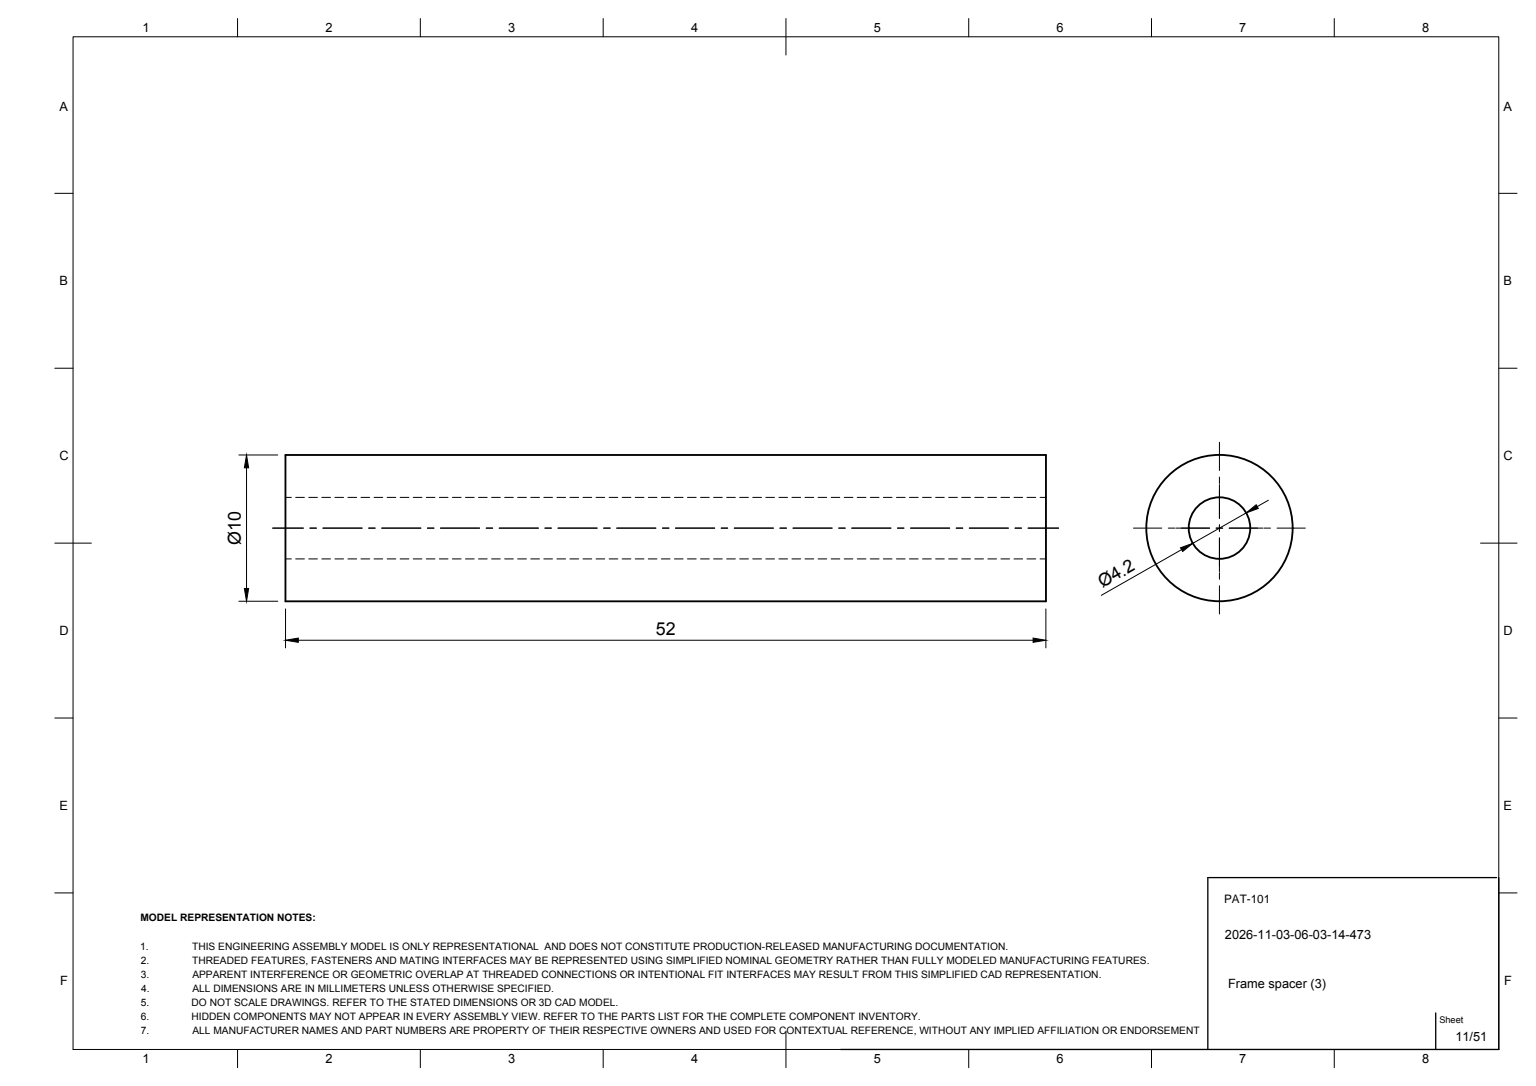
ISO-10303-21;
HEADER;
/* Generated by software containing ST-Developer
 * from STEP Tools, Inc. (www.steptools.com) 
 */

FILE_DESCRIPTION(
/* description */ ('Spur gear reduction stage 2-1 on bearing plates'),
/* implementation_level */ '2;1');

FILE_NAME(
/* name */ 'Frame spacer (3).step',
/* time_stamp */ '2026-10-28T03:22:07-07:00',
/* author */ (''),
/* organization */ (''),
/* preprocessor_version */ 'ST-DEVELOPER v20.2',
/* originating_system */ 'Autodesk Translation Framework v15.17.0.0',
/* authorisation */ '');

FILE_SCHEMA (('AUTOMOTIVE_DESIGN { 1 0 10303 214 3 1 1 }'));
ENDSEC;

DATA;
#10=MECHANICAL_DESIGN_GEOMETRIC_PRESENTATION_REPRESENTATION('',(#953),#53909);
#867=SHAPE_REPRESENTATION_RELATIONSHIP('SRR','None',#54094,#910);
#910=ADVANCED_BREP_SHAPE_REPRESENTATION('',(#1011),#53868);
#953=STYLED_ITEM('',(#54376),#1011);
#1011=MANIFOLD_SOLID_BREP('Body1',#11277);
#1138=FACE_BOUND('',#2322,.T.);
#1139=FACE_BOUND('',#2324,.T.);
#1278=PLANE('',#12011);
#1279=PLANE('',#12012);
#1593=FACE_OUTER_BOUND('',#2319,.T.);
#1594=FACE_OUTER_BOUND('',#2320,.T.);
#1595=FACE_OUTER_BOUND('',#2321,.T.);
#1596=FACE_OUTER_BOUND('',#2323,.T.);
#2319=EDGE_LOOP('',(#7724,#7725,#7726,#7727));
#2320=EDGE_LOOP('',(#7728,#7729,#7730,#7731));
#2321=EDGE_LOOP('',(#7732));
#2322=EDGE_LOOP('',(#7733));
#2323=EDGE_LOOP('',(#7734));
#2324=EDGE_LOOP('',(#7735));
#3063=LINE('',#16388,#3704);
#3064=LINE('',#16394,#3705);
#3704=VECTOR('',#13470,0.210000000000001);
#3705=VECTOR('',#13477,0.5);
#4359=CIRCLE('',#12006,0.210000000000001);
#4360=CIRCLE('',#12007,0.210000000000001);
#4361=CIRCLE('',#12009,0.5);
#4362=CIRCLE('',#12010,0.5);
#4908=VERTEX_POINT('',#16385);
#4909=VERTEX_POINT('',#16387);
#4910=VERTEX_POINT('',#16391);
#4911=VERTEX_POINT('',#16393);
#6004=EDGE_CURVE('',#4908,#4908,#4359,.T.);
#6005=EDGE_CURVE('',#4908,#4909,#3063,.T.);
#6006=EDGE_CURVE('',#4909,#4909,#4360,.T.);
#6007=EDGE_CURVE('',#4910,#4910,#4361,.T.);
#6008=EDGE_CURVE('',#4910,#4911,#3064,.T.);
#6009=EDGE_CURVE('',#4911,#4911,#4362,.T.);
#7724=ORIENTED_EDGE('',*,*,#6004,.F.);
#7725=ORIENTED_EDGE('',*,*,#6005,.T.);
#7726=ORIENTED_EDGE('',*,*,#6006,.T.);
#7727=ORIENTED_EDGE('',*,*,#6005,.F.);
#7728=ORIENTED_EDGE('',*,*,#6007,.F.);
#7729=ORIENTED_EDGE('',*,*,#6008,.T.);
#7730=ORIENTED_EDGE('',*,*,#6009,.T.);
#7731=ORIENTED_EDGE('',*,*,#6008,.F.);
#7732=ORIENTED_EDGE('',*,*,#6007,.T.);
#7733=ORIENTED_EDGE('',*,*,#6004,.T.);
#7734=ORIENTED_EDGE('',*,*,#6009,.F.);
#7735=ORIENTED_EDGE('',*,*,#6006,.F.);
#10470=CYLINDRICAL_SURFACE('',#12005,0.210000000000001);
#10471=CYLINDRICAL_SURFACE('',#12008,0.5);
#10713=ADVANCED_FACE('',(#1593),#10470,.F.);
#10714=ADVANCED_FACE('',(#1594),#10471,.T.);
#10715=ADVANCED_FACE('',(#1595,#1138),#1278,.T.);
#10716=ADVANCED_FACE('',(#1596,#1139),#1279,.F.);
#11277=CLOSED_SHELL('',(#10713,#10714,#10715,#10716));
#12004=AXIS2_PLACEMENT_3D('',#16383,#13464,#13465);
#12005=AXIS2_PLACEMENT_3D('',#16384,#13466,#13467);
#12006=AXIS2_PLACEMENT_3D('',#16386,#13468,#13469);
#12007=AXIS2_PLACEMENT_3D('',#16389,#13471,#13472);
#12008=AXIS2_PLACEMENT_3D('',#16390,#13473,#13474);
#12009=AXIS2_PLACEMENT_3D('',#16392,#13475,#13476);
#12010=AXIS2_PLACEMENT_3D('',#16395,#13478,#13479);
#12011=AXIS2_PLACEMENT_3D('',#16396,#13480,#13481);
#12012=AXIS2_PLACEMENT_3D('',#16397,#13482,#13483);
#13464=DIRECTION('axis',(0.,0.,1.));
#13465=DIRECTION('refdir',(1.,0.,0.));
#13466=DIRECTION('center_axis',(0.,1.,0.));
#13467=DIRECTION('ref_axis',(1.,0.,0.));
#13468=DIRECTION('center_axis',(0.,-1.,0.));
#13469=DIRECTION('ref_axis',(1.,0.,0.));
#13470=DIRECTION('',(0.,-1.,0.));
#13471=DIRECTION('center_axis',(0.,-1.,0.));
#13472=DIRECTION('ref_axis',(1.,0.,0.));
#13473=DIRECTION('center_axis',(0.,1.,0.));
#13474=DIRECTION('ref_axis',(1.,0.,0.));
#13475=DIRECTION('center_axis',(0.,1.,0.));
#13476=DIRECTION('ref_axis',(1.,0.,0.));
#13477=DIRECTION('',(0.,-1.,0.));
#13478=DIRECTION('center_axis',(0.,1.,0.));
#13479=DIRECTION('ref_axis',(1.,0.,0.));
#13480=DIRECTION('center_axis',(0.,1.,0.));
#13481=DIRECTION('ref_axis',(1.,0.,0.));
#13482=DIRECTION('center_axis',(0.,1.,0.));
#13483=DIRECTION('ref_axis',(1.,0.,0.));
#16383=CARTESIAN_POINT('',(0.,0.,0.));
#16384=CARTESIAN_POINT('Origin',(10.,-2.6,9.));
#16385=CARTESIAN_POINT('',(9.79,2.6,9.));
#16386=CARTESIAN_POINT('Origin',(10.,2.6,9.));
#16387=CARTESIAN_POINT('',(9.79,-2.6,9.));
#16388=CARTESIAN_POINT('',(9.79,-2.6,9.));
#16389=CARTESIAN_POINT('Origin',(10.,-2.6,9.));
#16390=CARTESIAN_POINT('Origin',(10.,-2.6,9.));
#16391=CARTESIAN_POINT('',(9.5,2.6,9.));
#16392=CARTESIAN_POINT('Origin',(10.,2.6,9.));
#16393=CARTESIAN_POINT('',(9.5,-2.6,9.));
#16394=CARTESIAN_POINT('',(9.5,-2.6,9.));
#16395=CARTESIAN_POINT('Origin',(10.,-2.6,9.));
#16396=CARTESIAN_POINT('Origin',(10.,2.6,9.));
#16397=CARTESIAN_POINT('Origin',(10.,-2.6,9.));
#53818=UNCERTAINTY_MEASURE_WITH_UNIT(LENGTH_MEASURE(0.001),#53910,
'DISTANCE_ACCURACY_VALUE',
'Maximum model space distance between geometric entities at asserted c
onnectivities');
#53859=UNCERTAINTY_MEASURE_WITH_UNIT(LENGTH_MEASURE(0.001),#53910,
'DISTANCE_ACCURACY_VALUE',
'Maximum model space distance between geometric entities at asserted c
onnectivities');
#53868=(
GEOMETRIC_REPRESENTATION_CONTEXT(3)
GLOBAL_UNCERTAINTY_ASSIGNED_CONTEXT((#53818))
GLOBAL_UNIT_ASSIGNED_CONTEXT((#53910,#53912,#53913))
REPRESENTATION_CONTEXT('','3D')
);
#53909=(
GEOMETRIC_REPRESENTATION_CONTEXT(3)
GLOBAL_UNCERTAINTY_ASSIGNED_CONTEXT((#53859))
GLOBAL_UNIT_ASSIGNED_CONTEXT((#53910,#53912,#53913))
REPRESENTATION_CONTEXT('','3D')
);
#53910=(
LENGTH_UNIT()
NAMED_UNIT(*)
SI_UNIT(.CENTI.,.METRE.)
);
#53912=(
NAMED_UNIT(*)
PLANE_ANGLE_UNIT()
SI_UNIT($,.RADIAN.)
);
#53913=(
NAMED_UNIT(*)
SI_UNIT($,.STERADIAN.)
SOLID_ANGLE_UNIT()
);
#53922=SHAPE_DEFINITION_REPRESENTATION(#53971,#54094);
#53971=PRODUCT_DEFINITION_SHAPE('',$,#54144);
#54094=SHAPE_REPRESENTATION('',(#12004),#53868);
#54135=PRODUCT_DEFINITION_CONTEXT('part definition',#54284,'design');
#54144=PRODUCT_DEFINITION('Frame spacer (3)','Frame spacer (3)',#54193,#54135);
#54193=PRODUCT_DEFINITION_FORMATION('',$,#54294);
#54284=APPLICATION_CONTEXT(
'Core Data for Automotive Mechanical Design Process');
#54285=PRODUCT_CONTEXT('part definition',#54284,'mechanical');
#54294=PRODUCT('Frame spacer (3)','Frame spacer (3)','Frame spacer (3)',(#54285));
#54370=COLOUR_RGB('Dark Blue',0.08,0.2,0.34);
#54371=FILL_AREA_STYLE_COLOUR('',#54370);
#54372=FILL_AREA_STYLE('',(#54371));
#54373=SURFACE_STYLE_FILL_AREA(#54372);
#54374=SURFACE_SIDE_STYLE('',(#54373));
#54375=SURFACE_STYLE_USAGE(.BOTH.,#54374);
#54376=PRESENTATION_STYLE_ASSIGNMENT((#54375));
ENDSEC;
END-ISO-10303-21;
